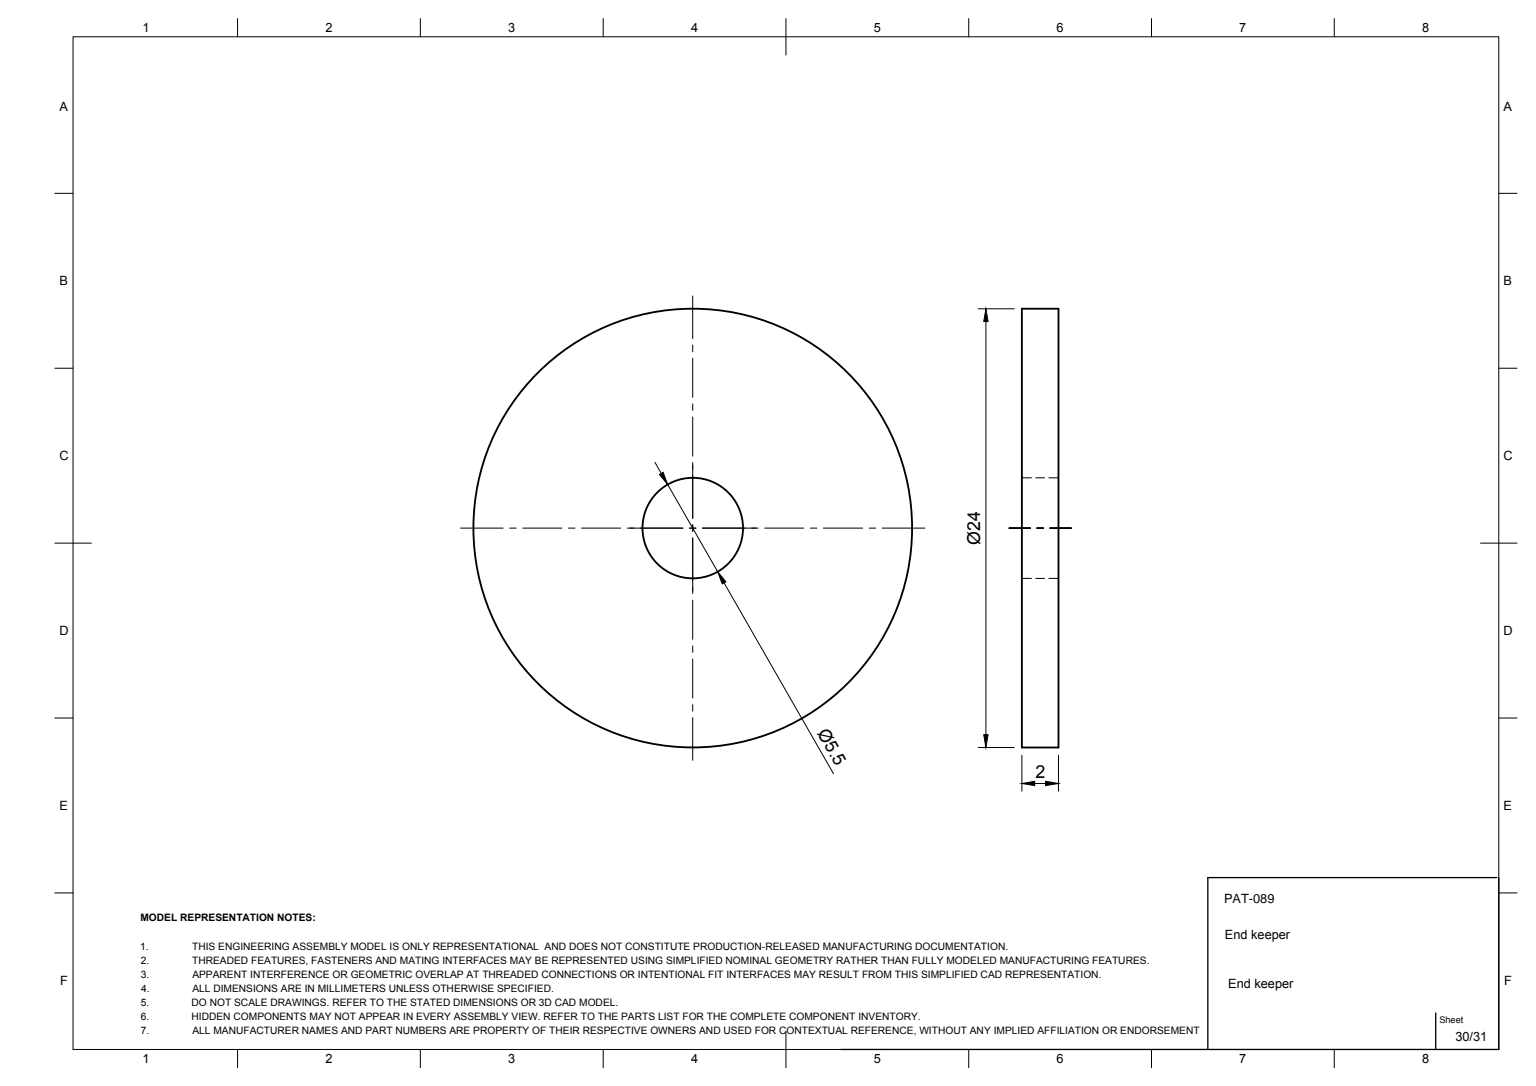
ISO-10303-21;
HEADER;
/* Generated by software containing ST-Developer
 * from STEP Tools, Inc. (www.steptools.com) 
 */

FILE_DESCRIPTION(
/* description */ ('Rotary union on bearing shaft'),
/* implementation_level */ '2;1');

FILE_NAME(
/* name */ 'End keeper.step',
/* time_stamp */ '2026-10-28T03:24:01-07:00',
/* author */ (''),
/* organization */ (''),
/* preprocessor_version */ 'ST-DEVELOPER v20.2',
/* originating_system */ 'Autodesk Translation Framework v15.17.0.0',
/* authorisation */ '');

FILE_SCHEMA (('AUTOMOTIVE_DESIGN { 1 0 10303 214 3 1 1 }'));
ENDSEC;

DATA;
#10=MECHANICAL_DESIGN_GEOMETRIC_PRESENTATION_REPRESENTATION('',(#343),#9448);
#281=SHAPE_REPRESENTATION_RELATIONSHIP('SRR','None',#9583,#308);
#308=ADVANCED_BREP_SHAPE_REPRESENTATION('',(#376),#9443);
#343=STYLED_ITEM('',(#9792),#376);
#376=MANIFOLD_SOLID_BREP('Body1',#4900);
#479=FACE_BOUND('',#1298,.T.);
#480=FACE_BOUND('',#1300,.T.);
#614=PLANE('',#5711);
#615=PLANE('',#5712);
#897=FACE_OUTER_BOUND('',#1295,.T.);
#898=FACE_OUTER_BOUND('',#1296,.T.);
#899=FACE_OUTER_BOUND('',#1297,.T.);
#900=FACE_OUTER_BOUND('',#1299,.T.);
#1295=EDGE_LOOP('',(#4243,#4244,#4245,#4246));
#1296=EDGE_LOOP('',(#4247,#4248,#4249,#4250));
#1297=EDGE_LOOP('',(#4251));
#1298=EDGE_LOOP('',(#4252));
#1299=EDGE_LOOP('',(#4253));
#1300=EDGE_LOOP('',(#4254));
#1587=LINE('',#9096,#1907);
#1588=LINE('',#9102,#1908);
#1907=VECTOR('',#7060,0.275);
#1908=VECTOR('',#7067,1.2);
#2229=CIRCLE('',#5706,0.275);
#2230=CIRCLE('',#5707,0.275);
#2231=CIRCLE('',#5709,1.2);
#2232=CIRCLE('',#5710,1.2);
#2585=VERTEX_POINT('',#9093);
#2586=VERTEX_POINT('',#9095);
#2587=VERTEX_POINT('',#9099);
#2588=VERTEX_POINT('',#9101);
#3149=EDGE_CURVE('',#2585,#2585,#2229,.T.);
#3150=EDGE_CURVE('',#2585,#2586,#1587,.T.);
#3151=EDGE_CURVE('',#2586,#2586,#2230,.T.);
#3152=EDGE_CURVE('',#2587,#2587,#2231,.T.);
#3153=EDGE_CURVE('',#2587,#2588,#1588,.T.);
#3154=EDGE_CURVE('',#2588,#2588,#2232,.T.);
#4243=ORIENTED_EDGE('',*,*,#3149,.F.);
#4244=ORIENTED_EDGE('',*,*,#3150,.T.);
#4245=ORIENTED_EDGE('',*,*,#3151,.T.);
#4246=ORIENTED_EDGE('',*,*,#3150,.F.);
#4247=ORIENTED_EDGE('',*,*,#3152,.F.);
#4248=ORIENTED_EDGE('',*,*,#3153,.T.);
#4249=ORIENTED_EDGE('',*,*,#3154,.T.);
#4250=ORIENTED_EDGE('',*,*,#3153,.F.);
#4251=ORIENTED_EDGE('',*,*,#3152,.T.);
#4252=ORIENTED_EDGE('',*,*,#3149,.T.);
#4253=ORIENTED_EDGE('',*,*,#3154,.F.);
#4254=ORIENTED_EDGE('',*,*,#3151,.F.);
#4561=CYLINDRICAL_SURFACE('',#5705,0.275);
#4562=CYLINDRICAL_SURFACE('',#5708,1.2);
#4810=ADVANCED_FACE('',(#897),#4561,.F.);
#4811=ADVANCED_FACE('',(#898),#4562,.T.);
#4812=ADVANCED_FACE('',(#899,#479),#614,.T.);
#4813=ADVANCED_FACE('',(#900,#480),#615,.F.);
#4900=CLOSED_SHELL('',(#4810,#4811,#4812,#4813));
#5704=AXIS2_PLACEMENT_3D('',#9091,#7054,#7055);
#5705=AXIS2_PLACEMENT_3D('',#9092,#7056,#7057);
#5706=AXIS2_PLACEMENT_3D('',#9094,#7058,#7059);
#5707=AXIS2_PLACEMENT_3D('',#9097,#7061,#7062);
#5708=AXIS2_PLACEMENT_3D('',#9098,#7063,#7064);
#5709=AXIS2_PLACEMENT_3D('',#9100,#7065,#7066);
#5710=AXIS2_PLACEMENT_3D('',#9103,#7068,#7069);
#5711=AXIS2_PLACEMENT_3D('',#9104,#7070,#7071);
#5712=AXIS2_PLACEMENT_3D('',#9105,#7072,#7073);
#7054=DIRECTION('axis',(0.,0.,1.));
#7055=DIRECTION('refdir',(1.,0.,0.));
#7056=DIRECTION('center_axis',(0.,1.,0.));
#7057=DIRECTION('ref_axis',(1.,0.,0.));
#7058=DIRECTION('center_axis',(0.,-1.,0.));
#7059=DIRECTION('ref_axis',(1.,0.,0.));
#7060=DIRECTION('',(0.,-1.,0.));
#7061=DIRECTION('center_axis',(0.,-1.,0.));
#7062=DIRECTION('ref_axis',(1.,0.,0.));
#7063=DIRECTION('center_axis',(0.,1.,0.));
#7064=DIRECTION('ref_axis',(1.,0.,0.));
#7065=DIRECTION('center_axis',(0.,1.,0.));
#7066=DIRECTION('ref_axis',(1.,0.,0.));
#7067=DIRECTION('',(0.,-1.,0.));
#7068=DIRECTION('center_axis',(0.,1.,0.));
#7069=DIRECTION('ref_axis',(1.,0.,0.));
#7070=DIRECTION('center_axis',(0.,1.,0.));
#7071=DIRECTION('ref_axis',(1.,0.,0.));
#7072=DIRECTION('center_axis',(0.,1.,0.));
#7073=DIRECTION('ref_axis',(1.,0.,0.));
#9091=CARTESIAN_POINT('',(0.,0.,0.));
#9092=CARTESIAN_POINT('Origin',(0.,10.,4.5));
#9093=CARTESIAN_POINT('',(-0.275,10.2,4.5));
#9094=CARTESIAN_POINT('Origin',(0.,10.2,4.5));
#9095=CARTESIAN_POINT('',(-0.275,10.,4.5));
#9096=CARTESIAN_POINT('',(-0.275,10.,4.5));
#9097=CARTESIAN_POINT('Origin',(0.,10.,4.5));
#9098=CARTESIAN_POINT('Origin',(0.,10.,4.5));
#9099=CARTESIAN_POINT('',(-1.2,10.2,4.5));
#9100=CARTESIAN_POINT('Origin',(0.,10.2,4.5));
#9101=CARTESIAN_POINT('',(-1.2,10.,4.5));
#9102=CARTESIAN_POINT('',(-1.2,10.,4.5));
#9103=CARTESIAN_POINT('Origin',(0.,10.,4.5));
#9104=CARTESIAN_POINT('Origin',(0.,10.2,4.5));
#9105=CARTESIAN_POINT('Origin',(0.,10.,4.5));
#9411=UNCERTAINTY_MEASURE_WITH_UNIT(LENGTH_MEASURE(0.001),#9449,
'DISTANCE_ACCURACY_VALUE',
'Maximum model space distance between geometric entities at asserted c
onnectivities');
#9416=UNCERTAINTY_MEASURE_WITH_UNIT(LENGTH_MEASURE(0.001),#9449,
'DISTANCE_ACCURACY_VALUE',
'Maximum model space distance between geometric entities at asserted c
onnectivities');
#9443=(
GEOMETRIC_REPRESENTATION_CONTEXT(3)
GLOBAL_UNCERTAINTY_ASSIGNED_CONTEXT((#9411))
GLOBAL_UNIT_ASSIGNED_CONTEXT((#9449,#9451,#9452))
REPRESENTATION_CONTEXT('','3D')
);
#9448=(
GEOMETRIC_REPRESENTATION_CONTEXT(3)
GLOBAL_UNCERTAINTY_ASSIGNED_CONTEXT((#9416))
GLOBAL_UNIT_ASSIGNED_CONTEXT((#9449,#9451,#9452))
REPRESENTATION_CONTEXT('','3D')
);
#9449=(
LENGTH_UNIT()
NAMED_UNIT(*)
SI_UNIT(.CENTI.,.METRE.)
);
#9451=(
NAMED_UNIT(*)
PLANE_ANGLE_UNIT()
SI_UNIT($,.RADIAN.)
);
#9452=(
NAMED_UNIT(*)
SI_UNIT($,.STERADIAN.)
SOLID_ANGLE_UNIT()
);
#9479=SHAPE_DEFINITION_REPRESENTATION(#9515,#9583);
#9515=PRODUCT_DEFINITION_SHAPE('',$,#9615);
#9583=SHAPE_REPRESENTATION('',(#5704),#9443);
#9588=PRODUCT_DEFINITION_CONTEXT('part definition',#9683,'design');
#9615=PRODUCT_DEFINITION('End keeper','End keeper',#9646,#9588);
#9646=PRODUCT_DEFINITION_FORMATION('',$,#9711);
#9683=APPLICATION_CONTEXT(
'Core Data for Automotive Mechanical Design Process');
#9684=PRODUCT_CONTEXT('part definition',#9683,'mechanical');
#9711=PRODUCT('End keeper','End keeper','End keeper',(#9684));
#9786=COLOUR_RGB('Off White',0.89,0.88,0.83);
#9787=FILL_AREA_STYLE_COLOUR('',#9786);
#9788=FILL_AREA_STYLE('',(#9787));
#9789=SURFACE_STYLE_FILL_AREA(#9788);
#9790=SURFACE_SIDE_STYLE('',(#9789));
#9791=SURFACE_STYLE_USAGE(.BOTH.,#9790);
#9792=PRESENTATION_STYLE_ASSIGNMENT((#9791));
ENDSEC;
END-ISO-10303-21;
